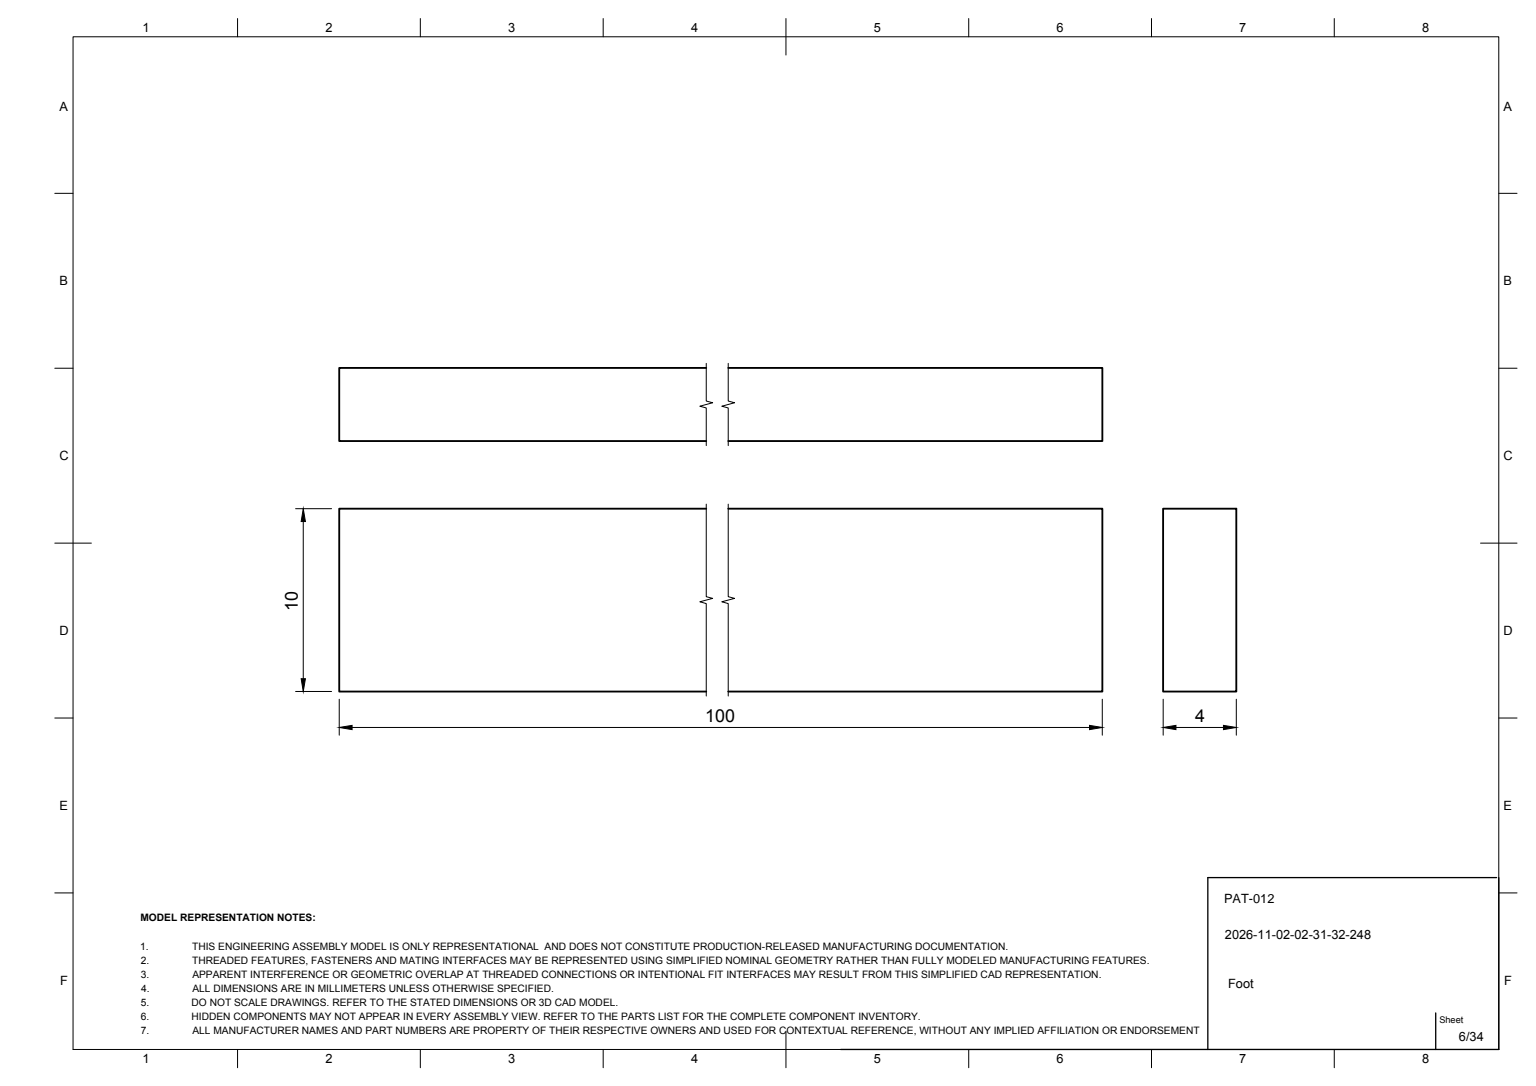
ISO-10303-21;
HEADER;
/* Generated by software containing ST-Developer
 * from STEP Tools, Inc. (www.steptools.com) 
 */

FILE_DESCRIPTION(
/* description */ ('Belt tensioner idler arm'),
/* implementation_level */ '2;1');

FILE_NAME(
/* name */ 'Foot.step',
/* time_stamp */ '2026-10-28T03:22:15-07:00',
/* author */ (''),
/* organization */ (''),
/* preprocessor_version */ 'ST-DEVELOPER v20.2',
/* originating_system */ 'Autodesk Translation Framework v15.17.0.0',
/* authorisation */ '');

FILE_SCHEMA (('AUTOMOTIVE_DESIGN { 1 0 10303 214 3 1 1 }'));
ENDSEC;

DATA;
#10=MECHANICAL_DESIGN_GEOMETRIC_PRESENTATION_REPRESENTATION('',(#448),#12779);
#380=SHAPE_REPRESENTATION_RELATIONSHIP('SRR','None',#12926,#414);
#414=ADVANCED_BREP_SHAPE_REPRESENTATION('',(#490),#12743);
#448=STYLED_ITEM('',(#13198),#490);
#490=MANIFOLD_SOLID_BREP('Body1',#6182);
#669=PLANE('',#6627);
#670=PLANE('',#6628);
#671=PLANE('',#6629);
#672=PLANE('',#6630);
#673=PLANE('',#6631);
#674=PLANE('',#6632);
#848=FACE_OUTER_BOUND('',#1225,.T.);
#849=FACE_OUTER_BOUND('',#1226,.T.);
#850=FACE_OUTER_BOUND('',#1227,.T.);
#851=FACE_OUTER_BOUND('',#1228,.T.);
#852=FACE_OUTER_BOUND('',#1229,.T.);
#853=FACE_OUTER_BOUND('',#1230,.T.);
#1225=EDGE_LOOP('',(#4140,#4141,#4142,#4143));
#1226=EDGE_LOOP('',(#4144,#4145,#4146,#4147));
#1227=EDGE_LOOP('',(#4148,#4149,#4150,#4151));
#1228=EDGE_LOOP('',(#4152,#4153,#4154,#4155));
#1229=EDGE_LOOP('',(#4156,#4157,#4158,#4159));
#1230=EDGE_LOOP('',(#4160,#4161,#4162,#4163));
#1724=LINE('',#9507,#2073);
#1725=LINE('',#9509,#2074);
#1726=LINE('',#9511,#2075);
#1727=LINE('',#9512,#2076);
#1728=LINE('',#9515,#2077);
#1729=LINE('',#9517,#2078);
#1730=LINE('',#9518,#2079);
#1731=LINE('',#9521,#2080);
#1732=LINE('',#9523,#2081);
#1733=LINE('',#9524,#2082);
#1734=LINE('',#9526,#2083);
#1735=LINE('',#9527,#2084);
#2073=VECTOR('',#7502,1.);
#2074=VECTOR('',#7503,1.);
#2075=VECTOR('',#7504,1.);
#2076=VECTOR('',#7505,1.);
#2077=VECTOR('',#7508,1.);
#2078=VECTOR('',#7509,1.);
#2079=VECTOR('',#7510,1.);
#2080=VECTOR('',#7513,1.);
#2081=VECTOR('',#7514,1.);
#2082=VECTOR('',#7515,1.);
#2083=VECTOR('',#7518,1.);
#2084=VECTOR('',#7519,1.);
#2787=VERTEX_POINT('',#9505);
#2788=VERTEX_POINT('',#9506);
#2789=VERTEX_POINT('',#9508);
#2790=VERTEX_POINT('',#9510);
#2791=VERTEX_POINT('',#9514);
#2792=VERTEX_POINT('',#9516);
#2793=VERTEX_POINT('',#9520);
#2794=VERTEX_POINT('',#9522);
#3325=EDGE_CURVE('',#2787,#2788,#1724,.T.);
#3326=EDGE_CURVE('',#2788,#2789,#1725,.T.);
#3327=EDGE_CURVE('',#2790,#2789,#1726,.T.);
#3328=EDGE_CURVE('',#2787,#2790,#1727,.T.);
#3329=EDGE_CURVE('',#2791,#2787,#1728,.T.);
#3330=EDGE_CURVE('',#2792,#2790,#1729,.T.);
#3331=EDGE_CURVE('',#2791,#2792,#1730,.T.);
#3332=EDGE_CURVE('',#2793,#2791,#1731,.T.);
#3333=EDGE_CURVE('',#2794,#2792,#1732,.T.);
#3334=EDGE_CURVE('',#2793,#2794,#1733,.T.);
#3335=EDGE_CURVE('',#2788,#2793,#1734,.T.);
#3336=EDGE_CURVE('',#2789,#2794,#1735,.T.);
#4140=ORIENTED_EDGE('',*,*,#3325,.T.);
#4141=ORIENTED_EDGE('',*,*,#3326,.T.);
#4142=ORIENTED_EDGE('',*,*,#3327,.F.);
#4143=ORIENTED_EDGE('',*,*,#3328,.F.);
#4144=ORIENTED_EDGE('',*,*,#3329,.T.);
#4145=ORIENTED_EDGE('',*,*,#3328,.T.);
#4146=ORIENTED_EDGE('',*,*,#3330,.F.);
#4147=ORIENTED_EDGE('',*,*,#3331,.F.);
#4148=ORIENTED_EDGE('',*,*,#3332,.T.);
#4149=ORIENTED_EDGE('',*,*,#3331,.T.);
#4150=ORIENTED_EDGE('',*,*,#3333,.F.);
#4151=ORIENTED_EDGE('',*,*,#3334,.F.);
#4152=ORIENTED_EDGE('',*,*,#3335,.T.);
#4153=ORIENTED_EDGE('',*,*,#3334,.T.);
#4154=ORIENTED_EDGE('',*,*,#3336,.F.);
#4155=ORIENTED_EDGE('',*,*,#3326,.F.);
#4156=ORIENTED_EDGE('',*,*,#3336,.T.);
#4157=ORIENTED_EDGE('',*,*,#3333,.T.);
#4158=ORIENTED_EDGE('',*,*,#3330,.T.);
#4159=ORIENTED_EDGE('',*,*,#3327,.T.);
#4160=ORIENTED_EDGE('',*,*,#3335,.F.);
#4161=ORIENTED_EDGE('',*,*,#3325,.F.);
#4162=ORIENTED_EDGE('',*,*,#3329,.F.);
#4163=ORIENTED_EDGE('',*,*,#3332,.F.);
#5825=ADVANCED_FACE('',(#848),#669,.T.);
#5826=ADVANCED_FACE('',(#849),#670,.T.);
#5827=ADVANCED_FACE('',(#850),#671,.T.);
#5828=ADVANCED_FACE('',(#851),#672,.T.);
#5829=ADVANCED_FACE('',(#852),#673,.T.);
#5830=ADVANCED_FACE('',(#853),#674,.F.);
#6182=CLOSED_SHELL('',(#5825,#5826,#5827,#5828,#5829,#5830));
#6626=AXIS2_PLACEMENT_3D('',#9503,#7498,#7499);
#6627=AXIS2_PLACEMENT_3D('',#9504,#7500,#7501);
#6628=AXIS2_PLACEMENT_3D('',#9513,#7506,#7507);
#6629=AXIS2_PLACEMENT_3D('',#9519,#7511,#7512);
#6630=AXIS2_PLACEMENT_3D('',#9525,#7516,#7517);
#6631=AXIS2_PLACEMENT_3D('',#9528,#7520,#7521);
#6632=AXIS2_PLACEMENT_3D('',#9529,#7522,#7523);
#7498=DIRECTION('axis',(0.,0.,1.));
#7499=DIRECTION('refdir',(1.,0.,0.));
#7500=DIRECTION('center_axis',(0.,1.,0.));
#7501=DIRECTION('ref_axis',(-1.,0.,0.));
#7502=DIRECTION('',(-1.,0.,0.));
#7503=DIRECTION('',(0.,0.,1.));
#7504=DIRECTION('',(-1.,0.,0.));
#7505=DIRECTION('',(0.,0.,1.));
#7506=DIRECTION('center_axis',(1.,0.,0.));
#7507=DIRECTION('ref_axis',(0.,1.,0.));
#7508=DIRECTION('',(0.,1.,0.));
#7509=DIRECTION('',(0.,1.,0.));
#7510=DIRECTION('',(0.,0.,1.));
#7511=DIRECTION('center_axis',(0.,-1.,0.));
#7512=DIRECTION('ref_axis',(1.,0.,0.));
#7513=DIRECTION('',(1.,0.,0.));
#7514=DIRECTION('',(1.,0.,0.));
#7515=DIRECTION('',(0.,0.,1.));
#7516=DIRECTION('center_axis',(-1.,0.,0.));
#7517=DIRECTION('ref_axis',(0.,-1.,0.));
#7518=DIRECTION('',(0.,-1.,0.));
#7519=DIRECTION('',(0.,-1.,0.));
#7520=DIRECTION('center_axis',(0.,0.,1.));
#7521=DIRECTION('ref_axis',(1.,0.,0.));
#7522=DIRECTION('center_axis',(0.,0.,1.));
#7523=DIRECTION('ref_axis',(1.,0.,0.));
#9503=CARTESIAN_POINT('',(0.,0.,0.));
#9504=CARTESIAN_POINT('Origin',(-2.,5.5,-1.4));
#9505=CARTESIAN_POINT('',(-2.,5.5,-1.4));
#9506=CARTESIAN_POINT('',(-3.,5.5,-1.4));
#9507=CARTESIAN_POINT('',(-2.,5.5,-1.4));
#9508=CARTESIAN_POINT('',(-3.,5.5,-1.));
#9509=CARTESIAN_POINT('',(-3.,5.5,-1.4));
#9510=CARTESIAN_POINT('',(-2.,5.5,-1.));
#9511=CARTESIAN_POINT('',(-2.,5.5,-1.));
#9512=CARTESIAN_POINT('',(-2.,5.5,-1.4));
#9513=CARTESIAN_POINT('Origin',(-2.,-4.5,-1.4));
#9514=CARTESIAN_POINT('',(-2.,-4.5,-1.4));
#9515=CARTESIAN_POINT('',(-2.,-4.5,-1.4));
#9516=CARTESIAN_POINT('',(-2.,-4.5,-1.));
#9517=CARTESIAN_POINT('',(-2.,-4.5,-1.));
#9518=CARTESIAN_POINT('',(-2.,-4.5,-1.4));
#9519=CARTESIAN_POINT('Origin',(-3.,-4.5,-1.4));
#9520=CARTESIAN_POINT('',(-3.,-4.5,-1.4));
#9521=CARTESIAN_POINT('',(-3.,-4.5,-1.4));
#9522=CARTESIAN_POINT('',(-3.,-4.5,-1.));
#9523=CARTESIAN_POINT('',(-3.,-4.5,-1.));
#9524=CARTESIAN_POINT('',(-3.,-4.5,-1.4));
#9525=CARTESIAN_POINT('Origin',(-3.,5.5,-1.4));
#9526=CARTESIAN_POINT('',(-3.,5.5,-1.4));
#9527=CARTESIAN_POINT('',(-3.,5.5,-1.));
#9528=CARTESIAN_POINT('Origin',(-2.5,0.5,-1.));
#9529=CARTESIAN_POINT('Origin',(-2.5,0.5,-1.4));
#12703=UNCERTAINTY_MEASURE_WITH_UNIT(LENGTH_MEASURE(0.001),#12780,
'DISTANCE_ACCURACY_VALUE',
'Maximum model space distance between geometric entities at asserted c
onnectivities');
#12739=UNCERTAINTY_MEASURE_WITH_UNIT(LENGTH_MEASURE(0.001),#12780,
'DISTANCE_ACCURACY_VALUE',
'Maximum model space distance between geometric entities at asserted c
onnectivities');
#12743=(
GEOMETRIC_REPRESENTATION_CONTEXT(3)
GLOBAL_UNCERTAINTY_ASSIGNED_CONTEXT((#12703))
GLOBAL_UNIT_ASSIGNED_CONTEXT((#12780,#12782,#12783))
REPRESENTATION_CONTEXT('','3D')
);
#12779=(
GEOMETRIC_REPRESENTATION_CONTEXT(3)
GLOBAL_UNCERTAINTY_ASSIGNED_CONTEXT((#12739))
GLOBAL_UNIT_ASSIGNED_CONTEXT((#12780,#12782,#12783))
REPRESENTATION_CONTEXT('','3D')
);
#12780=(
LENGTH_UNIT()
NAMED_UNIT(*)
SI_UNIT(.CENTI.,.METRE.)
);
#12782=(
NAMED_UNIT(*)
PLANE_ANGLE_UNIT()
SI_UNIT($,.RADIAN.)
);
#12783=(
NAMED_UNIT(*)
SI_UNIT($,.STERADIAN.)
SOLID_ANGLE_UNIT()
);
#12787=SHAPE_DEFINITION_REPRESENTATION(#12826,#12926);
#12826=PRODUCT_DEFINITION_SHAPE('',$,#12966);
#12926=SHAPE_REPRESENTATION('',(#6626),#12743);
#12962=PRODUCT_DEFINITION_CONTEXT('part definition',#13081,'design');
#12966=PRODUCT_DEFINITION('Foot','Foot',#13005,#12962);
#13005=PRODUCT_DEFINITION_FORMATION('',$,#13086);
#13081=APPLICATION_CONTEXT(
'Core Data for Automotive Mechanical Design Process');
#13082=PRODUCT_CONTEXT('part definition',#13081,'mechanical');
#13086=PRODUCT('Foot','Foot','Foot',(#13082));
#13192=COLOUR_RGB('Off White',0.89,0.88,0.83);
#13193=FILL_AREA_STYLE_COLOUR('',#13192);
#13194=FILL_AREA_STYLE('',(#13193));
#13195=SURFACE_STYLE_FILL_AREA(#13194);
#13196=SURFACE_SIDE_STYLE('',(#13195));
#13197=SURFACE_STYLE_USAGE(.BOTH.,#13196);
#13198=PRESENTATION_STYLE_ASSIGNMENT((#13197));
ENDSEC;
END-ISO-10303-21;
